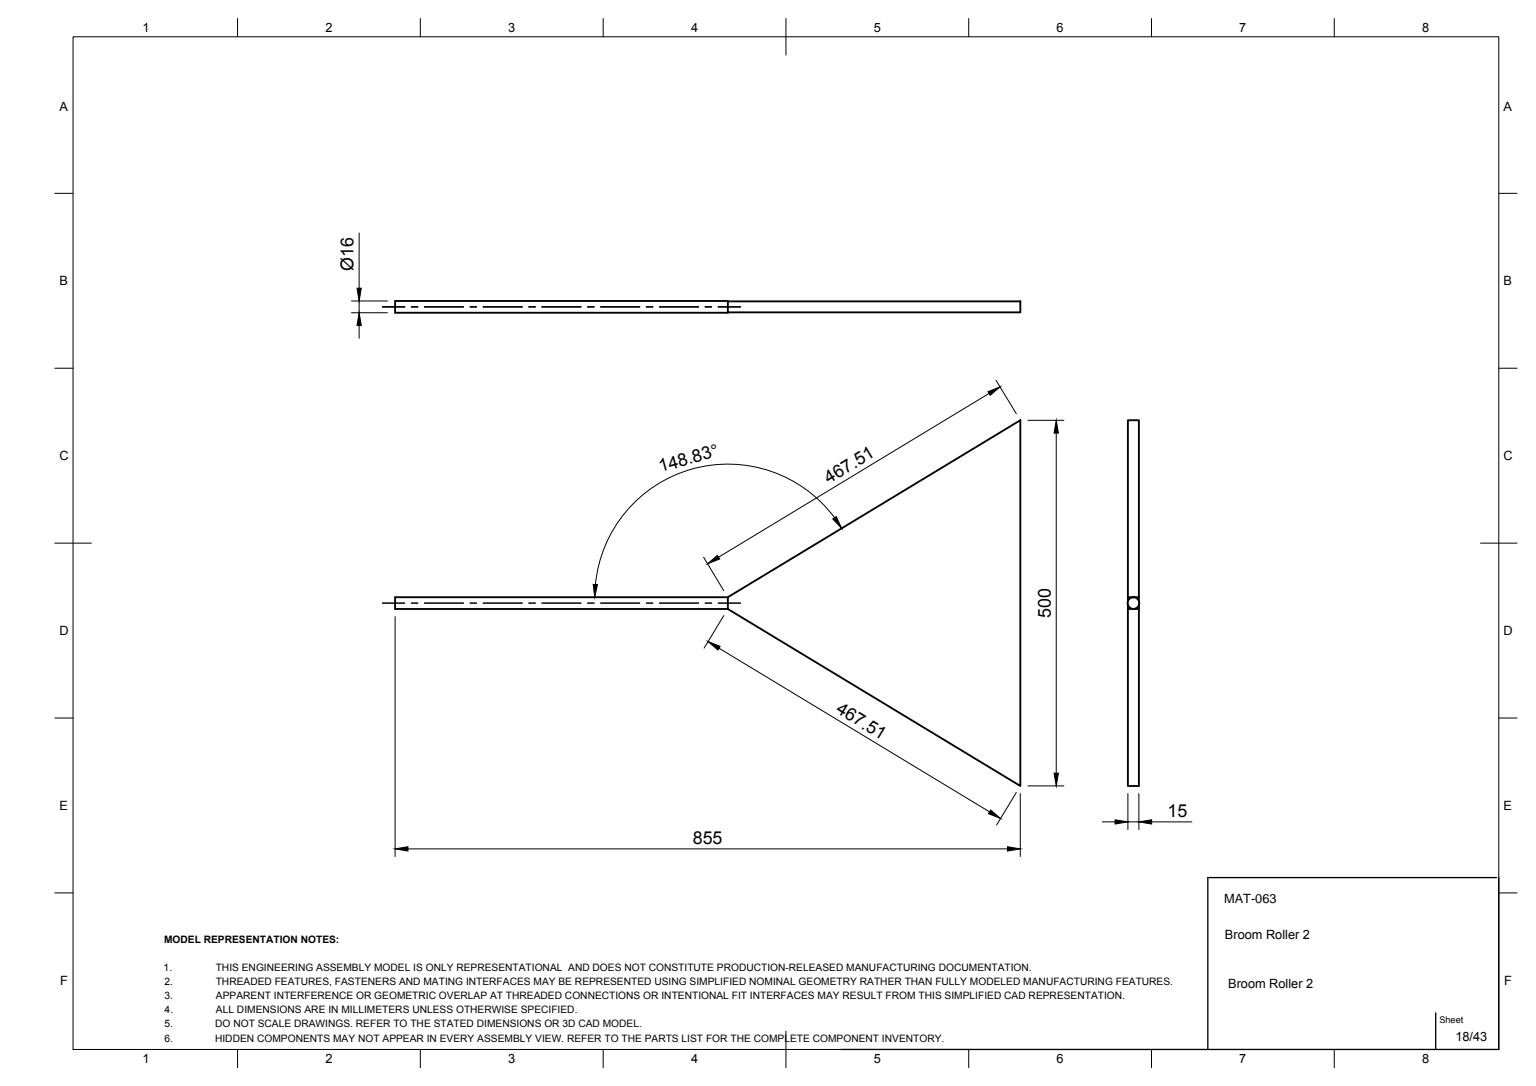
ISO-10303-21;
HEADER;
/* Generated by software containing ST-Developer
 * from STEP Tools, Inc. (www.steptools.com) 
 */

FILE_DESCRIPTION(
/* description */ (''),
/* implementation_level */ '2;1');

FILE_NAME(
/* name */ 'Broom Roller 2.step',
/* time_stamp */ '2026-10-24T09:43:01-07:00',
/* author */ (''),
/* organization */ (''),
/* preprocessor_version */ 'ST-DEVELOPER v20.2',
/* originating_system */ 'Autodesk Translation Framework v15.15.0.0',
/* authorisation */ '');

FILE_SCHEMA (('AUTOMOTIVE_DESIGN { 1 0 10303 214 3 1 1 }'));
ENDSEC;

DATA;
#10=MECHANICAL_DESIGN_GEOMETRIC_PRESENTATION_REPRESENTATION('',(#283),#11112);
#217=SHAPE_REPRESENTATION_RELATIONSHIP('SRR','None',#11241,#250);
#250=ADVANCED_BREP_SHAPE_REPRESENTATION('',(#316),#11086);
#283=STYLED_ITEM('',(#11426),#316);
#316=MANIFOLD_SOLID_BREP('Broom Roller 2',#6020);
#546=PLANE('',#6848);
#547=PLANE('',#6849);
#548=PLANE('',#6850);
#549=PLANE('',#6851);
#550=PLANE('',#6852);
#551=PLANE('',#6853);
#552=PLANE('',#6854);
#553=PLANE('',#6855);
#554=PLANE('',#6856);
#555=PLANE('',#6857);
#556=PLANE('',#6858);
#557=PLANE('',#6859);
#842=FACE_OUTER_BOUND('',#1280,.T.);
#843=FACE_OUTER_BOUND('',#1281,.T.);
#844=FACE_OUTER_BOUND('',#1282,.T.);
#845=FACE_OUTER_BOUND('',#1283,.T.);
#846=FACE_OUTER_BOUND('',#1284,.T.);
#847=FACE_OUTER_BOUND('',#1285,.T.);
#848=FACE_OUTER_BOUND('',#1286,.T.);
#849=FACE_OUTER_BOUND('',#1287,.T.);
#850=FACE_OUTER_BOUND('',#1288,.T.);
#851=FACE_OUTER_BOUND('',#1289,.T.);
#852=FACE_OUTER_BOUND('',#1290,.T.);
#853=FACE_OUTER_BOUND('',#1291,.T.);
#854=FACE_OUTER_BOUND('',#1292,.T.);
#1280=EDGE_LOOP('',(#4679,#4680,#4681,#4682,#4683,#4684,#4685,#4686,#4687,
#4688));
#1281=EDGE_LOOP('',(#4689));
#1282=EDGE_LOOP('',(#4690,#4691,#4692));
#1283=EDGE_LOOP('',(#4693,#4694,#4695));
#1284=EDGE_LOOP('',(#4696,#4697,#4698));
#1285=EDGE_LOOP('',(#4699,#4700));
#1286=EDGE_LOOP('',(#4701,#4702,#4703));
#1287=EDGE_LOOP('',(#4704,#4705,#4706));
#1288=EDGE_LOOP('',(#4707,#4708,#4709,#4710,#4711,#4712));
#1289=EDGE_LOOP('',(#4713,#4714,#4715,#4716,#4717));
#1290=EDGE_LOOP('',(#4718,#4719,#4720,#4721,#4722,#4723));
#1291=EDGE_LOOP('',(#4724,#4725,#4726,#4727,#4728));
#1292=EDGE_LOOP('',(#4729,#4730,#4731,#4732));
#1671=LINE('',#10111,#2030);
#1672=LINE('',#10120,#2031);
#1673=LINE('',#10123,#2032);
#1674=LINE('',#10124,#2033);
#1675=LINE('',#10127,#2034);
#1676=LINE('',#10128,#2035);
#1677=LINE('',#10130,#2036);
#1678=LINE('',#10133,#2037);
#1679=LINE('',#10134,#2038);
#1680=LINE('',#10137,#2039);
#1681=LINE('',#10138,#2040);
#1682=LINE('',#10141,#2041);
#1683=LINE('',#10143,#2042);
#1684=LINE('',#10144,#2043);
#1685=LINE('',#10147,#2044);
#1686=LINE('',#10148,#2045);
#1687=LINE('',#10151,#2046);
#1688=LINE('',#10152,#2047);
#1689=LINE('',#10154,#2048);
#2030=VECTOR('',#8247,0.00799999961340774);
#2031=VECTOR('',#8260,0.01);
#2032=VECTOR('',#8263,0.01);
#2033=VECTOR('',#8264,0.01);
#2034=VECTOR('',#8267,0.01);
#2035=VECTOR('',#8268,0.01);
#2036=VECTOR('',#8271,0.01);
#2037=VECTOR('',#8274,0.01);
#2038=VECTOR('',#8275,0.01);
#2039=VECTOR('',#8278,0.01);
#2040=VECTOR('',#8279,0.01);
#2041=VECTOR('',#8282,0.01);
#2042=VECTOR('',#8283,0.01);
#2043=VECTOR('',#8284,0.01);
#2044=VECTOR('',#8287,0.01);
#2045=VECTOR('',#8288,0.01);
#2046=VECTOR('',#8291,0.01);
#2047=VECTOR('',#8292,0.01);
#2048=VECTOR('',#8295,0.01);
#2526=CIRCLE('',#6840,0.00799999961340774);
#2527=CIRCLE('',#6841,0.00799999961340774);
#2528=CIRCLE('',#6842,0.00799999961340774);
#2529=CIRCLE('',#6843,0.00799999961340774);
#2530=CIRCLE('',#6844,0.00799999961340774);
#2531=CIRCLE('',#6845,0.00799999961340774);
#2532=CIRCLE('',#6846,0.00799999961340774);
#2533=CIRCLE('',#6847,0.00799999961340774);
#2912=VERTEX_POINT('',#10101);
#2913=VERTEX_POINT('',#10102);
#2914=VERTEX_POINT('',#10104);
#2915=VERTEX_POINT('',#10106);
#2916=VERTEX_POINT('',#10108);
#2917=VERTEX_POINT('',#10110);
#2918=VERTEX_POINT('',#10113);
#2919=VERTEX_POINT('',#10115);
#2920=VERTEX_POINT('',#10122);
#2921=VERTEX_POINT('',#10126);
#2922=VERTEX_POINT('',#10132);
#2923=VERTEX_POINT('',#10136);
#2924=VERTEX_POINT('',#10140);
#2925=VERTEX_POINT('',#10142);
#2926=VERTEX_POINT('',#10146);
#2927=VERTEX_POINT('',#10150);
#3543=EDGE_CURVE('',#2912,#2913,#2526,.F.);
#3544=EDGE_CURVE('',#2913,#2914,#2527,.F.);
#3545=EDGE_CURVE('',#2914,#2915,#2528,.F.);
#3546=EDGE_CURVE('',#2915,#2916,#2529,.F.);
#3547=EDGE_CURVE('',#2916,#2917,#1671,.T.);
#3548=EDGE_CURVE('',#2917,#2917,#2530,.T.);
#3549=EDGE_CURVE('',#2916,#2918,#2531,.F.);
#3550=EDGE_CURVE('',#2918,#2919,#2532,.F.);
#3551=EDGE_CURVE('',#2919,#2912,#2533,.F.);
#3552=EDGE_CURVE('',#2915,#2918,#1672,.T.);
#3553=EDGE_CURVE('',#2920,#2919,#1673,.T.);
#3554=EDGE_CURVE('',#2918,#2920,#1674,.T.);
#3555=EDGE_CURVE('',#2921,#2912,#1675,.T.);
#3556=EDGE_CURVE('',#2919,#2921,#1676,.T.);
#3557=EDGE_CURVE('',#2912,#2913,#1677,.T.);
#3558=EDGE_CURVE('',#2922,#2914,#1678,.T.);
#3559=EDGE_CURVE('',#2913,#2922,#1679,.T.);
#3560=EDGE_CURVE('',#2923,#2915,#1680,.T.);
#3561=EDGE_CURVE('',#2914,#2923,#1681,.T.);
#3562=EDGE_CURVE('',#2924,#2923,#1682,.T.);
#3563=EDGE_CURVE('',#2925,#2924,#1683,.T.);
#3564=EDGE_CURVE('',#2920,#2925,#1684,.T.);
#3565=EDGE_CURVE('',#2926,#2925,#1685,.T.);
#3566=EDGE_CURVE('',#2921,#2926,#1686,.T.);
#3567=EDGE_CURVE('',#2926,#2927,#1687,.T.);
#3568=EDGE_CURVE('',#2927,#2922,#1688,.T.);
#3569=EDGE_CURVE('',#2927,#2924,#1689,.T.);
#4679=ORIENTED_EDGE('',*,*,#3543,.T.);
#4680=ORIENTED_EDGE('',*,*,#3544,.T.);
#4681=ORIENTED_EDGE('',*,*,#3545,.T.);
#4682=ORIENTED_EDGE('',*,*,#3546,.T.);
#4683=ORIENTED_EDGE('',*,*,#3547,.T.);
#4684=ORIENTED_EDGE('',*,*,#3548,.T.);
#4685=ORIENTED_EDGE('',*,*,#3547,.F.);
#4686=ORIENTED_EDGE('',*,*,#3549,.T.);
#4687=ORIENTED_EDGE('',*,*,#3550,.T.);
#4688=ORIENTED_EDGE('',*,*,#3551,.T.);
#4689=ORIENTED_EDGE('',*,*,#3548,.F.);
#4690=ORIENTED_EDGE('',*,*,#3552,.T.);
#4691=ORIENTED_EDGE('',*,*,#3549,.F.);
#4692=ORIENTED_EDGE('',*,*,#3546,.F.);
#4693=ORIENTED_EDGE('',*,*,#3553,.T.);
#4694=ORIENTED_EDGE('',*,*,#3550,.F.);
#4695=ORIENTED_EDGE('',*,*,#3554,.T.);
#4696=ORIENTED_EDGE('',*,*,#3555,.T.);
#4697=ORIENTED_EDGE('',*,*,#3551,.F.);
#4698=ORIENTED_EDGE('',*,*,#3556,.T.);
#4699=ORIENTED_EDGE('',*,*,#3557,.T.);
#4700=ORIENTED_EDGE('',*,*,#3543,.F.);
#4701=ORIENTED_EDGE('',*,*,#3558,.T.);
#4702=ORIENTED_EDGE('',*,*,#3544,.F.);
#4703=ORIENTED_EDGE('',*,*,#3559,.T.);
#4704=ORIENTED_EDGE('',*,*,#3560,.T.);
#4705=ORIENTED_EDGE('',*,*,#3545,.F.);
#4706=ORIENTED_EDGE('',*,*,#3561,.T.);
#4707=ORIENTED_EDGE('',*,*,#3562,.F.);
#4708=ORIENTED_EDGE('',*,*,#3563,.F.);
#4709=ORIENTED_EDGE('',*,*,#3564,.F.);
#4710=ORIENTED_EDGE('',*,*,#3554,.F.);
#4711=ORIENTED_EDGE('',*,*,#3552,.F.);
#4712=ORIENTED_EDGE('',*,*,#3560,.F.);
#4713=ORIENTED_EDGE('',*,*,#3553,.F.);
#4714=ORIENTED_EDGE('',*,*,#3564,.T.);
#4715=ORIENTED_EDGE('',*,*,#3565,.F.);
#4716=ORIENTED_EDGE('',*,*,#3566,.F.);
#4717=ORIENTED_EDGE('',*,*,#3556,.F.);
#4718=ORIENTED_EDGE('',*,*,#3567,.T.);
#4719=ORIENTED_EDGE('',*,*,#3568,.T.);
#4720=ORIENTED_EDGE('',*,*,#3559,.F.);
#4721=ORIENTED_EDGE('',*,*,#3557,.F.);
#4722=ORIENTED_EDGE('',*,*,#3555,.F.);
#4723=ORIENTED_EDGE('',*,*,#3566,.T.);
#4724=ORIENTED_EDGE('',*,*,#3562,.T.);
#4725=ORIENTED_EDGE('',*,*,#3561,.F.);
#4726=ORIENTED_EDGE('',*,*,#3558,.F.);
#4727=ORIENTED_EDGE('',*,*,#3568,.F.);
#4728=ORIENTED_EDGE('',*,*,#3569,.T.);
#4729=ORIENTED_EDGE('',*,*,#3565,.T.);
#4730=ORIENTED_EDGE('',*,*,#3563,.T.);
#4731=ORIENTED_EDGE('',*,*,#3569,.F.);
#4732=ORIENTED_EDGE('',*,*,#3567,.F.);
#5570=CYLINDRICAL_SURFACE('',#6839,0.00799999961340774);
#5815=ADVANCED_FACE('',(#842),#5570,.T.);
#5816=ADVANCED_FACE('',(#843),#546,.F.);
#5817=ADVANCED_FACE('',(#844),#547,.T.);
#5818=ADVANCED_FACE('',(#845),#548,.T.);
#5819=ADVANCED_FACE('',(#846),#549,.T.);
#5820=ADVANCED_FACE('',(#847),#550,.T.);
#5821=ADVANCED_FACE('',(#848),#551,.T.);
#5822=ADVANCED_FACE('',(#849),#552,.T.);
#5823=ADVANCED_FACE('',(#850),#553,.F.);
#5824=ADVANCED_FACE('',(#851),#554,.F.);
#5825=ADVANCED_FACE('',(#852),#555,.T.);
#5826=ADVANCED_FACE('',(#853),#556,.T.);
#5827=ADVANCED_FACE('',(#854),#557,.F.);
#6020=CLOSED_SHELL('',(#5815,#5816,#5817,#5818,#5819,#5820,#5821,#5822,
#5823,#5824,#5825,#5826,#5827));
#6838=AXIS2_PLACEMENT_3D('',#10099,#8235,#8236);
#6839=AXIS2_PLACEMENT_3D('',#10100,#8237,#8238);
#6840=AXIS2_PLACEMENT_3D('',#10103,#8239,#8240);
#6841=AXIS2_PLACEMENT_3D('',#10105,#8241,#8242);
#6842=AXIS2_PLACEMENT_3D('',#10107,#8243,#8244);
#6843=AXIS2_PLACEMENT_3D('',#10109,#8245,#8246);
#6844=AXIS2_PLACEMENT_3D('',#10112,#8248,#8249);
#6845=AXIS2_PLACEMENT_3D('',#10114,#8250,#8251);
#6846=AXIS2_PLACEMENT_3D('',#10116,#8252,#8253);
#6847=AXIS2_PLACEMENT_3D('',#10117,#8254,#8255);
#6848=AXIS2_PLACEMENT_3D('',#10118,#8256,#8257);
#6849=AXIS2_PLACEMENT_3D('',#10119,#8258,#8259);
#6850=AXIS2_PLACEMENT_3D('',#10121,#8261,#8262);
#6851=AXIS2_PLACEMENT_3D('',#10125,#8265,#8266);
#6852=AXIS2_PLACEMENT_3D('',#10129,#8269,#8270);
#6853=AXIS2_PLACEMENT_3D('',#10131,#8272,#8273);
#6854=AXIS2_PLACEMENT_3D('',#10135,#8276,#8277);
#6855=AXIS2_PLACEMENT_3D('',#10139,#8280,#8281);
#6856=AXIS2_PLACEMENT_3D('',#10145,#8285,#8286);
#6857=AXIS2_PLACEMENT_3D('',#10149,#8289,#8290);
#6858=AXIS2_PLACEMENT_3D('',#10153,#8293,#8294);
#6859=AXIS2_PLACEMENT_3D('',#10155,#8296,#8297);
#8235=DIRECTION('axis',(0.,0.,1.));
#8236=DIRECTION('refdir',(1.,0.,0.));
#8237=DIRECTION('center_axis',(0.,-0.99219341162106,0.124708596078064));
#8238=DIRECTION('ref_axis',(0.,-0.124708596078064,-0.99219341162106));
#8239=DIRECTION('center_axis',(0.,-0.99219341162106,0.124708596078064));
#8240=DIRECTION('ref_axis',(0.,-0.124708596078064,-0.99219341162106));
#8241=DIRECTION('center_axis',(0.,-0.99219341162106,0.124708596078064));
#8242=DIRECTION('ref_axis',(0.,-0.124708596078064,-0.99219341162106));
#8243=DIRECTION('center_axis',(0.,-0.99219341162106,0.124708596078064));
#8244=DIRECTION('ref_axis',(0.,-0.124708596078064,-0.99219341162106));
#8245=DIRECTION('center_axis',(0.,-0.99219341162106,0.124708596078064));
#8246=DIRECTION('ref_axis',(0.,-0.124708596078064,-0.99219341162106));
#8247=DIRECTION('',(0.,0.99219341162106,-0.124708596078064));
#8248=DIRECTION('center_axis',(0.,-0.99219341162106,0.124708596078064));
#8249=DIRECTION('ref_axis',(0.,-0.124708596078064,-0.99219341162106));
#8250=DIRECTION('center_axis',(0.,-0.99219341162106,0.124708596078064));
#8251=DIRECTION('ref_axis',(0.,-0.124708596078064,-0.99219341162106));
#8252=DIRECTION('center_axis',(0.,-0.99219341162106,0.124708596078064));
#8253=DIRECTION('ref_axis',(0.,-0.124708596078064,-0.99219341162106));
#8254=DIRECTION('center_axis',(0.,-0.99219341162106,0.124708596078064));
#8255=DIRECTION('ref_axis',(0.,-0.124708596078064,-0.99219341162106));
#8256=DIRECTION('center_axis',(-3.56161599407301E-15,-0.992193416380086,
0.124708558214796));
#8257=DIRECTION('ref_axis',(5.41945887256173E-32,-0.124708558214796,-0.992193416380086));
#8258=DIRECTION('center_axis',(9.14782393218023E-15,-0.992193507035639,
0.124707836948281));
#8259=DIRECTION('ref_axis',(-3.40310025056597E-32,-0.124707836948281,-0.992193507035639));
#8260=DIRECTION('',(1.,0.,0.));
#8261=DIRECTION('center_axis',(-2.03678483080916E-15,0.992193402544911,
-0.124708668288743));
#8262=DIRECTION('ref_axis',(4.13177645825422E-32,0.124708668288743,0.992193402544911));
#8263=DIRECTION('',(3.27320801842311E-8,-0.124708648640395,-0.992193405014509));
#8264=DIRECTION('',(1.,0.,0.));
#8265=DIRECTION('center_axis',(-8.81386107600706E-16,0.992193416883257,
-0.124708554211516));
#8266=DIRECTION('ref_axis',(7.20809393353264E-33,0.124708554211516,0.992193416883257));
#8267=DIRECTION('',(-1.,0.,0.));
#8268=DIRECTION('',(-1.81892028111732E-8,-0.124708565130038,-0.992193415510911));
#8269=DIRECTION('center_axis',(1.3069838162107E-15,-0.992193291960435,0.124709548105651));
#8270=DIRECTION('ref_axis',(-6.81953595921427E-33,-0.124709548105651,-0.992193291960435));
#8271=DIRECTION('',(-1.,0.,0.));
#8272=DIRECTION('center_axis',(-8.75485997098923E-16,0.992193416883257,
-0.124708554211516));
#8273=DIRECTION('ref_axis',(5.40831068588944E-33,0.124708554211516,0.992193416883257));
#8274=DIRECTION('',(-1.81892161321154E-8,0.124708565130016,0.992193415510914));
#8275=DIRECTION('',(-1.,0.,0.));
#8276=DIRECTION('center_axis',(-2.04304168492322E-15,0.992193402544911,
-0.124708668288743));
#8277=DIRECTION('ref_axis',(-3.57454093922697E-33,0.124708668288743,0.992193402544911));
#8278=DIRECTION('',(1.,0.,0.));
#8279=DIRECTION('',(3.27320408114478E-8,0.124708648640324,0.992193405014518));
#8280=DIRECTION('center_axis',(-4.36194494519598E-17,-0.124708594908011,
-0.992193411768124));
#8281=DIRECTION('ref_axis',(2.29865079049834E-34,0.992193411768124,-0.124708594908011));
#8282=DIRECTION('',(0.517637880127419,0.848920488901183,-0.106700649393379));
#8283=DIRECTION('',(-1.,0.,0.));
#8284=DIRECTION('',(0.517637880127419,-0.848920488901183,0.106700649393379));
#8285=DIRECTION('center_axis',(-0.855599804264349,-0.513596894340652,0.0645538927288335));
#8286=DIRECTION('ref_axis',(0.514670382381903,-0.857388125354478,2.04082986758841E-17));
#8287=DIRECTION('',(-6.44853564777329E-9,0.124708601376938,0.992193410955046));
#8288=DIRECTION('',(0.51763788012742,-0.848920488901183,0.106700649393376));
#8289=DIRECTION('center_axis',(3.7067617295265E-17,-0.124708594908011,-0.992193411768124));
#8290=DIRECTION('ref_axis',(8.52848234808661E-35,0.992193411768124,-0.124708594908011));
#8291=DIRECTION('',(-1.,0.,0.));
#8292=DIRECTION('',(0.517637880127419,0.848920488901183,-0.106700649393379));
#8293=DIRECTION('center_axis',(-0.855599804264349,0.513596894340652,-0.0645538927288335));
#8294=DIRECTION('ref_axis',(-0.514670382381903,-0.857388125354478,2.04082986758841E-17));
#8295=DIRECTION('',(6.44853327929739E-9,0.124708601376938,0.992193410955046));
#8296=DIRECTION('center_axis',(-1.20013551743046E-17,0.992193410955045,
-0.12470860137694));
#8297=DIRECTION('ref_axis',(4.64258476562535E-35,0.12470860137694,0.992193410955045));
#10099=CARTESIAN_POINT('',(0.,0.,0.));
#10100=CARTESIAN_POINT('Origin',(0.,0.305351296,1.105611887));
#10101=CARTESIAN_POINT('',(0.00278388211169927,-0.147032020331956,1.15491284800427));
#10102=CARTESIAN_POINT('',(-0.00278388211169927,-0.147032020331956,1.15491284800427));
#10103=CARTESIAN_POINT('Origin',(0.,-0.146096706241833,1.16235429820977));
#10104=CARTESIAN_POINT('',(-0.00800000000069301,-0.14609670602179,1.16235429794207));
#10105=CARTESIAN_POINT('Origin',(0.,-0.146096706241833,1.16235429820977));
#10106=CARTESIAN_POINT('',(-0.0027838802685275,-0.145161391367063,1.16979574904614));
#10107=CARTESIAN_POINT('Origin',(0.,-0.146096706241833,1.16235429820977));
#10108=CARTESIAN_POINT('',(-9.79717391973985E-19,-0.14509903752142,1.17029184511916));
#10109=CARTESIAN_POINT('Origin',(0.,-0.146096706241833,1.16235429820977));
#10110=CARTESIAN_POINT('',(-9.79717391973985E-19,0.306348965440833,1.11354943381884));
#10111=CARTESIAN_POINT('',(-9.79717391973985E-19,0.306348964720413,1.11354943390939));
#10112=CARTESIAN_POINT('Origin',(0.,0.30535129672042,1.10561188690945));
#10113=CARTESIAN_POINT('',(0.00278388026853193,-0.145161391367063,1.16979574904614));
#10114=CARTESIAN_POINT('Origin',(0.,-0.146096706241833,1.16235429820977));
#10115=CARTESIAN_POINT('',(0.00800000000069306,-0.146096706021879,1.16235429794136));
#10116=CARTESIAN_POINT('Origin',(0.,-0.146096706241833,1.16235429820977));
#10117=CARTESIAN_POINT('Origin',(0.,-0.146096706241833,1.16235429820977));
#10118=CARTESIAN_POINT('Origin',(-1.99493199737333E-19,0.3053512965,1.105611887));
#10119=CARTESIAN_POINT('Origin',(-2.16840434497101E-21,-0.145130214061639,
1.17004379721066));
#10120=CARTESIAN_POINT('',(-0.00278388206046948,-0.145161391,1.169795749));
#10121=CARTESIAN_POINT('Origin',(0.0053919408556245,-0.145629048554537,
1.16607502335495));
#10122=CARTESIAN_POINT('',(0.00800000019173051,-0.145161390945555,1.16979574899316));
#10123=CARTESIAN_POINT('',(0.0080000001755413,-0.145161390894627,1.16979574898676));
#10124=CARTESIAN_POINT('',(0.00278388206046948,-0.145161391,1.169795749));
#10125=CARTESIAN_POINT('Origin',(0.0053919408556245,-0.146564362942481,
1.15863357314803));
#10126=CARTESIAN_POINT('',(0.00800000023881122,-0.147032019932316,1.15491284799148));
#10127=CARTESIAN_POINT('',(0.008,-0.14703202,1.154912848));
#10128=CARTESIAN_POINT('',(0.00800000035492486,-0.146096705717927,1.16235429790316));
#10129=CARTESIAN_POINT('Origin',(-2.16840434497101E-21,-0.147063197435379,
1.15466479929232));
#10130=CARTESIAN_POINT('',(0.00278388206047103,-0.14703202,1.154912848));
#10131=CARTESIAN_POINT('Origin',(-0.00539194085562444,-0.146564362942481,
1.15863357314803));
#10132=CARTESIAN_POINT('',(-0.00800000023876324,-0.147032019932289,1.15491284799148));
#10133=CARTESIAN_POINT('',(-0.00800000021850583,-0.147032019868836,1.15491284798351));
#10134=CARTESIAN_POINT('',(-0.00278388206047102,-0.14703202,1.154912848));
#10135=CARTESIAN_POINT('Origin',(-0.00539194085562444,-0.145629048554537,
1.16607502335495));
#10136=CARTESIAN_POINT('',(-0.00800000019173049,-0.145161390945555,1.16979574899316));
#10137=CARTESIAN_POINT('',(-0.00799999999999999,-0.145161391,1.169795749));
#10138=CARTESIAN_POINT('',(-0.00800000042103161,-0.146096705826252,1.16235429791749));
#10139=CARTESIAN_POINT('Origin',(-8.88178419700125E-18,-0.3436000735,1.194737468));
#10140=CARTESIAN_POINT('',(-0.249999999778211,-0.542038756006933,1.21967918700087));
#10141=CARTESIAN_POINT('',(-0.2499999997114,-0.542038755954343,1.21967918699426));
#10142=CARTESIAN_POINT('',(0.249999999778211,-0.542038756006933,1.21967918700087));
#10143=CARTESIAN_POINT('',(0.249999999800629,-0.542038756,1.219679187));
#10144=CARTESIAN_POINT('',(0.00800000019883055,-0.145161390932821,1.16979574899156));
#10145=CARTESIAN_POINT('Origin',(0.129,-0.344535388,1.18729601725));
#10146=CARTESIAN_POINT('',(0.249999999858746,-0.543909385010705,1.20479628600136));
#10147=CARTESIAN_POINT('',(0.249999999902924,-0.543909384930022,1.20479628655675));
#10148=CARTESIAN_POINT('',(0.00800000026765782,-0.147032019949447,1.15491284799364));
#10149=CARTESIAN_POINT('Origin',(-8.88178419700125E-18,-0.3454707025,1.17985456699999));
#10150=CARTESIAN_POINT('',(-0.249999999858735,-0.543909385010698,1.20479628600136));
#10151=CARTESIAN_POINT('',(0.249999999800629,-0.543909385000001,1.20479628599999));
#10152=CARTESIAN_POINT('',(-0.249999999754365,-0.543909384928553,1.20479628599101));
#10153=CARTESIAN_POINT('Origin',(-0.129,-0.344535388,1.18729601725));
#10154=CARTESIAN_POINT('',(-0.249999999902924,-0.543909384930022,1.20479628655675));
#10155=CARTESIAN_POINT('Origin',(-8.88178419700125E-18,-0.5429740705,1.2122377365));
#11047=UNCERTAINTY_MEASURE_WITH_UNIT(LENGTH_MEASURE(1.E-5),#11113,
'DISTANCE_ACCURACY_VALUE',
'Maximum model space distance between geometric entities at asserted c
onnectivities');
#11073=UNCERTAINTY_MEASURE_WITH_UNIT(LENGTH_MEASURE(1.E-5),#11113,
'DISTANCE_ACCURACY_VALUE',
'Maximum model space distance between geometric entities at asserted c
onnectivities');
#11086=(
GEOMETRIC_REPRESENTATION_CONTEXT(3)
GLOBAL_UNCERTAINTY_ASSIGNED_CONTEXT((#11047))
GLOBAL_UNIT_ASSIGNED_CONTEXT((#11113,#11114,#11115))
REPRESENTATION_CONTEXT('','3D')
);
#11112=(
GEOMETRIC_REPRESENTATION_CONTEXT(3)
GLOBAL_UNCERTAINTY_ASSIGNED_CONTEXT((#11073))
GLOBAL_UNIT_ASSIGNED_CONTEXT((#11113,#11114,#11115))
REPRESENTATION_CONTEXT('','3D')
);
#11113=(
LENGTH_UNIT()
NAMED_UNIT(*)
SI_UNIT($,.METRE.)
);
#11114=(
NAMED_UNIT(*)
PLANE_ANGLE_UNIT()
SI_UNIT($,.RADIAN.)
);
#11115=(
NAMED_UNIT(*)
SI_UNIT($,.STERADIAN.)
SOLID_ANGLE_UNIT()
);
#11128=SHAPE_DEFINITION_REPRESENTATION(#11166,#11241);
#11166=PRODUCT_DEFINITION_SHAPE('',$,#11280);
#11241=SHAPE_REPRESENTATION('',(#6838),#11086);
#11267=PRODUCT_DEFINITION_CONTEXT('part definition',#11383,'design');
#11280=PRODUCT_DEFINITION('Broom Roller 2','Broom Roller 2',#11318,#11267);
#11318=PRODUCT_DEFINITION_FORMATION('',$,#11397);
#11383=APPLICATION_CONTEXT(
'Core Data for Automotive Mechanical Design Process');
#11384=PRODUCT_CONTEXT('part definition',#11383,'mechanical');
#11397=PRODUCT('Broom Roller 2','Broom Roller 2',
'broom_and_roller__ DE     6147',(#11384));
#11426=PRESENTATION_STYLE_ASSIGNMENT((#11430));
#11430=SURFACE_STYLE_USAGE(.BOTH.,#11434);
#11434=SURFACE_SIDE_STYLE('',(#11438));
#11438=SURFACE_STYLE_FILL_AREA(#11442);
#11442=FILL_AREA_STYLE('Opaque(202,209,238)',(#11446));
#11446=FILL_AREA_STYLE_COLOUR('Opaque(202,209,238)',#11450);
#11450=COLOUR_RGB('Opaque(202,209,238)',0.792156862745098,0.819607843137255,
0.933333333333333);
ENDSEC;
END-ISO-10303-21;
